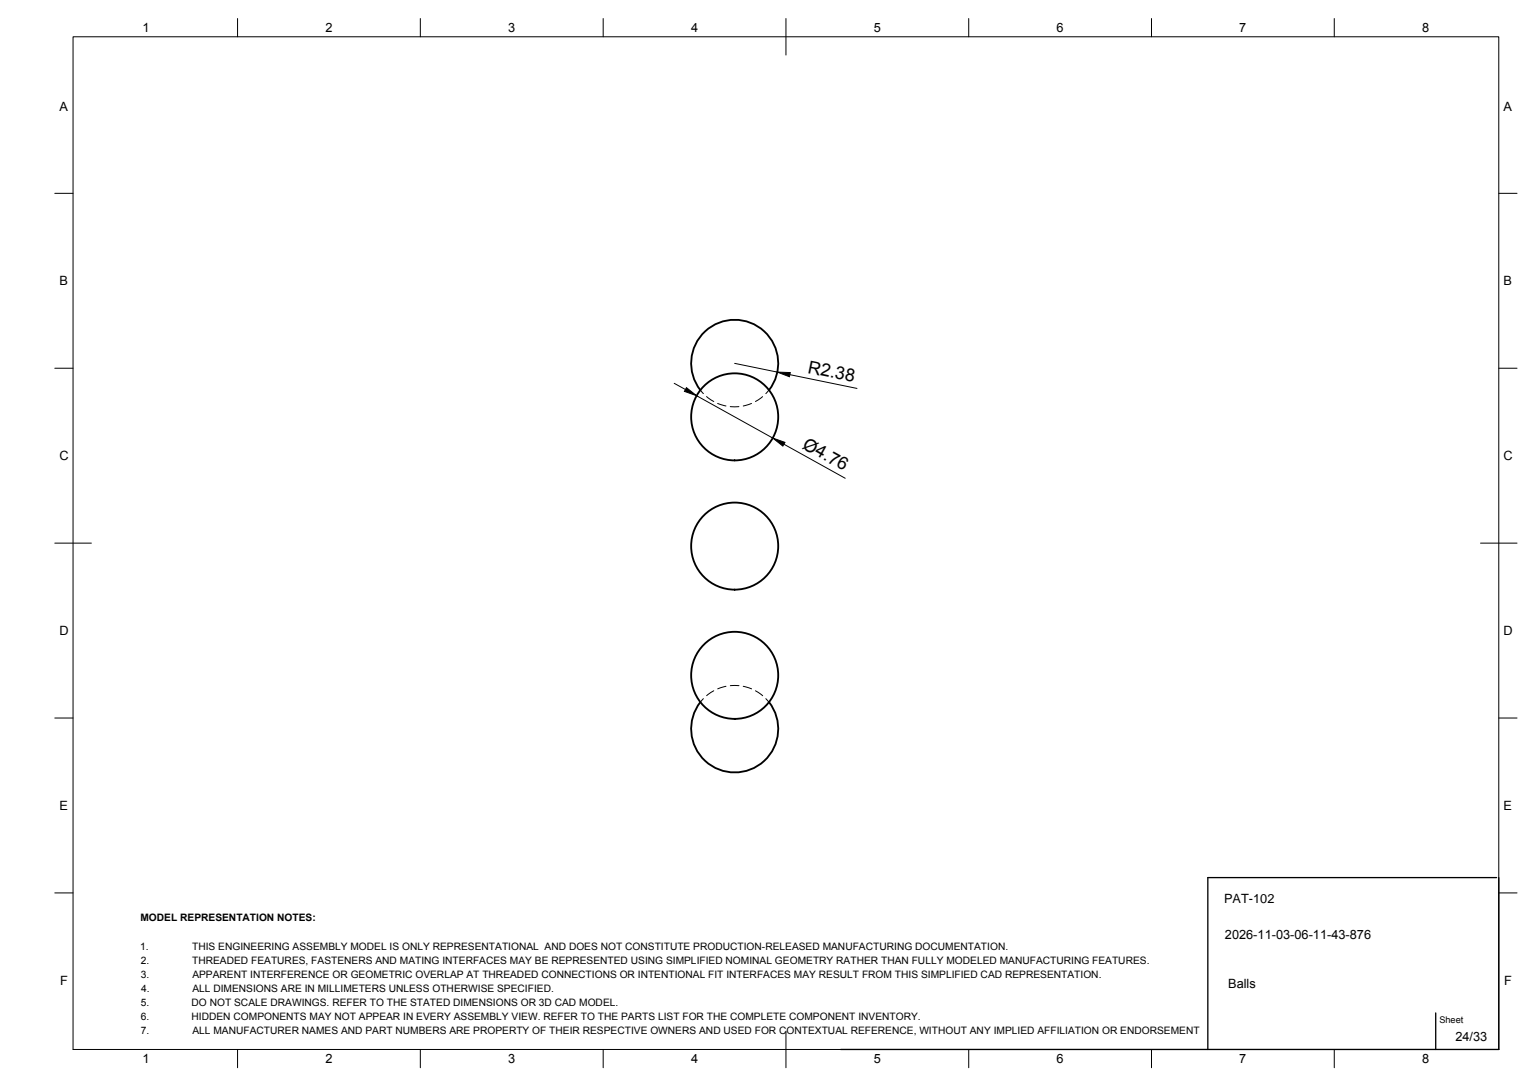
ISO-10303-21;
HEADER;
/* Generated by software containing ST-Developer
 * from STEP Tools, Inc. (www.steptools.com) 
 */

FILE_DESCRIPTION(
/* description */ ('Swing-away clamp arm'),
/* implementation_level */ '2;1');

FILE_NAME(
/* name */ 'Balls.step',
/* time_stamp */ '2026-10-28T03:26:03-07:00',
/* author */ (''),
/* organization */ (''),
/* preprocessor_version */ 'ST-DEVELOPER v20.2',
/* originating_system */ 'Autodesk Translation Framework v15.17.0.0',
/* authorisation */ '');

FILE_SCHEMA (('AUTOMOTIVE_DESIGN { 1 0 10303 214 3 1 1 }'));
ENDSEC;

DATA;
#10=MECHANICAL_DESIGN_GEOMETRIC_PRESENTATION_REPRESENTATION('',(#309,#310,#311,#312,#313,#314,#315,#316),#10627);
#11=SPHERICAL_SURFACE('',#5621,0.23815);
#12=SPHERICAL_SURFACE('',#5623,0.23815);
#13=SPHERICAL_SURFACE('',#5625,0.23815);
#14=SPHERICAL_SURFACE('',#5627,0.23815);
#15=SPHERICAL_SURFACE('',#5629,0.23815);
#16=SPHERICAL_SURFACE('',#5631,0.23815);
#17=SPHERICAL_SURFACE('',#5633,0.23815);
#18=SPHERICAL_SURFACE('',#5635,0.23815);
#257=SHAPE_REPRESENTATION_RELATIONSHIP('SRR','None',#10757,#283);
#283=ADVANCED_BREP_SHAPE_REPRESENTATION('',(#342,#343,#344,#345,#346,#347,
#348,#349),#10616);
#309=STYLED_ITEM('',(#10965),#342);
#310=STYLED_ITEM('',(#10965),#343);
#311=STYLED_ITEM('',(#10965),#344);
#312=STYLED_ITEM('',(#10965),#345);
#313=STYLED_ITEM('',(#10965),#346);
#314=STYLED_ITEM('',(#10965),#347);
#315=STYLED_ITEM('',(#10965),#348);
#316=STYLED_ITEM('',(#10965),#349);
#342=MANIFOLD_SOLID_BREP('Body1',#4916);
#343=MANIFOLD_SOLID_BREP('Body2',#4917);
#344=MANIFOLD_SOLID_BREP('Body3',#4918);
#345=MANIFOLD_SOLID_BREP('Body4',#4919);
#346=MANIFOLD_SOLID_BREP('Body5',#4920);
#347=MANIFOLD_SOLID_BREP('Body6',#4921);
#348=MANIFOLD_SOLID_BREP('Body7',#4922);
#349=MANIFOLD_SOLID_BREP('Body8',#4923);
#839=FACE_OUTER_BOUND('',#1224,.T.);
#840=FACE_OUTER_BOUND('',#1225,.T.);
#841=FACE_OUTER_BOUND('',#1226,.T.);
#842=FACE_OUTER_BOUND('',#1227,.T.);
#843=FACE_OUTER_BOUND('',#1228,.T.);
#844=FACE_OUTER_BOUND('',#1229,.T.);
#845=FACE_OUTER_BOUND('',#1230,.T.);
#846=FACE_OUTER_BOUND('',#1231,.T.);
#1224=EDGE_LOOP('',(#4105,#4106));
#1225=EDGE_LOOP('',(#4107,#4108));
#1226=EDGE_LOOP('',(#4109,#4110));
#1227=EDGE_LOOP('',(#4111,#4112));
#1228=EDGE_LOOP('',(#4113,#4114));
#1229=EDGE_LOOP('',(#4115,#4116));
#1230=EDGE_LOOP('',(#4117,#4118));
#1231=EDGE_LOOP('',(#4119,#4120));
#2161=CIRCLE('',#5622,0.23815);
#2162=CIRCLE('',#5624,0.23815);
#2163=CIRCLE('',#5626,0.23815);
#2164=CIRCLE('',#5628,0.23815);
#2165=CIRCLE('',#5630,0.23815);
#2166=CIRCLE('',#5632,0.23815);
#2167=CIRCLE('',#5634,0.23815);
#2168=CIRCLE('',#5636,0.23815);
#2534=VERTEX_POINT('',#9744);
#2535=VERTEX_POINT('',#9745);
#2536=VERTEX_POINT('',#9748);
#2537=VERTEX_POINT('',#9749);
#2538=VERTEX_POINT('',#9752);
#2539=VERTEX_POINT('',#9753);
#2540=VERTEX_POINT('',#9756);
#2541=VERTEX_POINT('',#9757);
#2542=VERTEX_POINT('',#9760);
#2543=VERTEX_POINT('',#9761);
#2544=VERTEX_POINT('',#9764);
#2545=VERTEX_POINT('',#9765);
#2546=VERTEX_POINT('',#9768);
#2547=VERTEX_POINT('',#9769);
#2548=VERTEX_POINT('',#9772);
#2549=VERTEX_POINT('',#9773);
#3085=EDGE_CURVE('',#2534,#2535,#2161,.T.);
#3086=EDGE_CURVE('',#2536,#2537,#2162,.T.);
#3087=EDGE_CURVE('',#2538,#2539,#2163,.T.);
#3088=EDGE_CURVE('',#2540,#2541,#2164,.T.);
#3089=EDGE_CURVE('',#2542,#2543,#2165,.T.);
#3090=EDGE_CURVE('',#2544,#2545,#2166,.T.);
#3091=EDGE_CURVE('',#2546,#2547,#2167,.T.);
#3092=EDGE_CURVE('',#2548,#2549,#2168,.T.);
#4105=ORIENTED_EDGE('',*,*,#3085,.T.);
#4106=ORIENTED_EDGE('',*,*,#3085,.F.);
#4107=ORIENTED_EDGE('',*,*,#3086,.T.);
#4108=ORIENTED_EDGE('',*,*,#3086,.F.);
#4109=ORIENTED_EDGE('',*,*,#3087,.T.);
#4110=ORIENTED_EDGE('',*,*,#3087,.F.);
#4111=ORIENTED_EDGE('',*,*,#3088,.T.);
#4112=ORIENTED_EDGE('',*,*,#3088,.F.);
#4113=ORIENTED_EDGE('',*,*,#3089,.T.);
#4114=ORIENTED_EDGE('',*,*,#3089,.F.);
#4115=ORIENTED_EDGE('',*,*,#3090,.T.);
#4116=ORIENTED_EDGE('',*,*,#3090,.F.);
#4117=ORIENTED_EDGE('',*,*,#3091,.T.);
#4118=ORIENTED_EDGE('',*,*,#3091,.F.);
#4119=ORIENTED_EDGE('',*,*,#3092,.T.);
#4120=ORIENTED_EDGE('',*,*,#3092,.F.);
#4794=ADVANCED_FACE('',(#839),#11,.T.);
#4795=ADVANCED_FACE('',(#840),#12,.T.);
#4796=ADVANCED_FACE('',(#841),#13,.T.);
#4797=ADVANCED_FACE('',(#842),#14,.T.);
#4798=ADVANCED_FACE('',(#843),#15,.T.);
#4799=ADVANCED_FACE('',(#844),#16,.T.);
#4800=ADVANCED_FACE('',(#845),#17,.T.);
#4801=ADVANCED_FACE('',(#846),#18,.T.);
#4916=CLOSED_SHELL('',(#4794));
#4917=CLOSED_SHELL('',(#4795));
#4918=CLOSED_SHELL('',(#4796));
#4919=CLOSED_SHELL('',(#4797));
#4920=CLOSED_SHELL('',(#4798));
#4921=CLOSED_SHELL('',(#4799));
#4922=CLOSED_SHELL('',(#4800));
#4923=CLOSED_SHELL('',(#4801));
#5620=AXIS2_PLACEMENT_3D('',#9742,#6909,#6910);
#5621=AXIS2_PLACEMENT_3D('',#9743,#6911,#6912);
#5622=AXIS2_PLACEMENT_3D('',#9746,#6913,#6914);
#5623=AXIS2_PLACEMENT_3D('',#9747,#6915,#6916);
#5624=AXIS2_PLACEMENT_3D('',#9750,#6917,#6918);
#5625=AXIS2_PLACEMENT_3D('',#9751,#6919,#6920);
#5626=AXIS2_PLACEMENT_3D('',#9754,#6921,#6922);
#5627=AXIS2_PLACEMENT_3D('',#9755,#6923,#6924);
#5628=AXIS2_PLACEMENT_3D('',#9758,#6925,#6926);
#5629=AXIS2_PLACEMENT_3D('',#9759,#6927,#6928);
#5630=AXIS2_PLACEMENT_3D('',#9762,#6929,#6930);
#5631=AXIS2_PLACEMENT_3D('',#9763,#6931,#6932);
#5632=AXIS2_PLACEMENT_3D('',#9766,#6933,#6934);
#5633=AXIS2_PLACEMENT_3D('',#9767,#6935,#6936);
#5634=AXIS2_PLACEMENT_3D('',#9770,#6937,#6938);
#5635=AXIS2_PLACEMENT_3D('',#9771,#6939,#6940);
#5636=AXIS2_PLACEMENT_3D('',#9774,#6941,#6942);
#6909=DIRECTION('axis',(0.,0.,1.));
#6910=DIRECTION('refdir',(1.,0.,0.));
#6911=DIRECTION('center_axis',(0.,0.,1.));
#6912=DIRECTION('ref_axis',(1.,0.,0.));
#6913=DIRECTION('center_axis',(1.22464679914735E-16,-1.,0.));
#6914=DIRECTION('ref_axis',(-1.,-1.22464679914735E-16,0.));
#6915=DIRECTION('center_axis',(0.707106781186548,0.,0.707106781186548));
#6916=DIRECTION('ref_axis',(0.707106781186548,0.,-0.707106781186548));
#6917=DIRECTION('center_axis',(8.65956056235494E-17,-1.,-8.65956056235493E-17));
#6918=DIRECTION('ref_axis',(-0.707106781186547,-1.22464679914735E-16,0.707106781186547));
#6919=DIRECTION('center_axis',(1.,0.,0.));
#6920=DIRECTION('ref_axis',(6.12323399573676E-17,0.,-1.));
#6921=DIRECTION('center_axis',(7.49879891330929E-33,-1.,-1.22464679914735E-16));
#6922=DIRECTION('ref_axis',(-6.12323399573676E-17,-1.22464679914735E-16,
1.));
#6923=DIRECTION('center_axis',(0.707106781186548,0.,-0.707106781186548));
#6924=DIRECTION('ref_axis',(-0.707106781186548,0.,-0.707106781186548));
#6925=DIRECTION('center_axis',(-8.65956056235493E-17,-1.,-8.65956056235494E-17));
#6926=DIRECTION('ref_axis',(0.707106781186547,-1.22464679914735E-16,0.707106781186547));
#6927=DIRECTION('center_axis',(0.,0.,-1.));
#6928=DIRECTION('ref_axis',(-1.,0.,-1.22464679914735E-16));
#6929=DIRECTION('center_axis',(-1.22464679914735E-16,-1.,-1.49975978266186E-32));
#6930=DIRECTION('ref_axis',(1.,-1.22464679914735E-16,1.22464679914735E-16));
#6931=DIRECTION('center_axis',(-0.707106781186547,0.,-0.707106781186548));
#6932=DIRECTION('ref_axis',(-0.707106781186548,0.,0.707106781186547));
#6933=DIRECTION('center_axis',(-8.65956056235493E-17,-1.,8.65956056235493E-17));
#6934=DIRECTION('ref_axis',(0.707106781186548,-1.22464679914735E-16,-0.707106781186547));
#6935=DIRECTION('center_axis',(-1.,0.,0.));
#6936=DIRECTION('ref_axis',(-1.83697019872103E-16,0.,1.));
#6937=DIRECTION('center_axis',(-2.24963967399279E-32,-1.,1.22464679914735E-16));
#6938=DIRECTION('ref_axis',(1.83697019872103E-16,-1.22464679914735E-16,
-1.));
#6939=DIRECTION('center_axis',(-0.707106781186548,0.,0.707106781186548));
#6940=DIRECTION('ref_axis',(0.707106781186547,0.,0.707106781186548));
#6941=DIRECTION('center_axis',(8.65956056235493E-17,-1.,8.65956056235493E-17));
#6942=DIRECTION('ref_axis',(-0.707106781186547,-1.22464679914735E-16,-0.707106781186548));
#9742=CARTESIAN_POINT('',(0.,0.,0.));
#9743=CARTESIAN_POINT('Origin',(1.,0.,0.));
#9744=CARTESIAN_POINT('',(1.,-1.78583896120461E-33,0.23815));
#9745=CARTESIAN_POINT('',(1.,-1.78583896120461E-33,-0.23815));
#9746=CARTESIAN_POINT('Origin',(1.,0.,0.));
#9747=CARTESIAN_POINT('Origin',(0.707106781186548,0.,-0.707106781186547));
#9748=CARTESIAN_POINT('',(0.875504261126124,-1.78583896120461E-33,-0.538709301246971));
#9749=CARTESIAN_POINT('',(0.538709301246971,-1.78583896120461E-33,-0.875504261126124));
#9750=CARTESIAN_POINT('Origin',(0.707106781186548,0.,-0.707106781186547));
#9751=CARTESIAN_POINT('Origin',(6.12323399573677E-17,0.,-1.));
#9752=CARTESIAN_POINT('',(0.23815,-1.78583896120461E-33,-1.));
#9753=CARTESIAN_POINT('',(-0.23815,-1.78583896120461E-33,-1.));
#9754=CARTESIAN_POINT('Origin',(6.12323399573677E-17,0.,-1.));
#9755=CARTESIAN_POINT('Origin',(-0.707106781186547,0.,-0.707106781186548));
#9756=CARTESIAN_POINT('',(-0.538709301246971,-1.78583896120461E-33,-0.875504261126124));
#9757=CARTESIAN_POINT('',(-0.875504261126124,-1.78583896120461E-33,-0.538709301246971));
#9758=CARTESIAN_POINT('Origin',(-0.707106781186547,0.,-0.707106781186548));
#9759=CARTESIAN_POINT('Origin',(-1.,0.,-1.22464679914735E-16));
#9760=CARTESIAN_POINT('',(-1.,-1.78583896120461E-33,-0.23815));
#9761=CARTESIAN_POINT('',(-1.,-1.78583896120461E-33,0.23815));
#9762=CARTESIAN_POINT('Origin',(-1.,0.,-1.22464679914735E-16));
#9763=CARTESIAN_POINT('Origin',(-0.707106781186548,0.,0.707106781186547));
#9764=CARTESIAN_POINT('',(-0.875504261126124,-7.94881478324376E-33,0.538709301246971));
#9765=CARTESIAN_POINT('',(-0.538709301246971,4.37713686083455E-33,0.875504261126124));
#9766=CARTESIAN_POINT('Origin',(-0.707106781186548,0.,0.707106781186547));
#9767=CARTESIAN_POINT('Origin',(-1.83697019872103E-16,0.,1.));
#9768=CARTESIAN_POINT('',(-0.23815,-1.78583896120461E-33,1.));
#9769=CARTESIAN_POINT('',(0.23815,-1.78583896120461E-33,1.));
#9770=CARTESIAN_POINT('Origin',(-1.83697019872103E-16,0.,1.));
#9771=CARTESIAN_POINT('Origin',(0.707106781186547,0.,0.707106781186548));
#9772=CARTESIAN_POINT('',(0.538709301246971,-4.86732687222419E-33,0.875504261126124));
#9773=CARTESIAN_POINT('',(0.875504261126124,1.29564894981497E-33,0.538709301246971));
#9774=CARTESIAN_POINT('Origin',(0.707106781186547,0.,0.707106781186548));
#10584=UNCERTAINTY_MEASURE_WITH_UNIT(LENGTH_MEASURE(0.001),#10628,
'DISTANCE_ACCURACY_VALUE',
'Maximum model space distance between geometric entities at asserted c
onnectivities');
#10595=UNCERTAINTY_MEASURE_WITH_UNIT(LENGTH_MEASURE(0.001),#10628,
'DISTANCE_ACCURACY_VALUE',
'Maximum model space distance between geometric entities at asserted c
onnectivities');
#10616=(
GEOMETRIC_REPRESENTATION_CONTEXT(3)
GLOBAL_UNCERTAINTY_ASSIGNED_CONTEXT((#10584))
GLOBAL_UNIT_ASSIGNED_CONTEXT((#10628,#10630,#10631))
REPRESENTATION_CONTEXT('','3D')
);
#10627=(
GEOMETRIC_REPRESENTATION_CONTEXT(3)
GLOBAL_UNCERTAINTY_ASSIGNED_CONTEXT((#10595))
GLOBAL_UNIT_ASSIGNED_CONTEXT((#10628,#10630,#10631))
REPRESENTATION_CONTEXT('','3D')
);
#10628=(
LENGTH_UNIT()
NAMED_UNIT(*)
SI_UNIT(.CENTI.,.METRE.)
);
#10630=(
NAMED_UNIT(*)
PLANE_ANGLE_UNIT()
SI_UNIT($,.RADIAN.)
);
#10631=(
NAMED_UNIT(*)
SI_UNIT($,.STERADIAN.)
SOLID_ANGLE_UNIT()
);
#10652=SHAPE_DEFINITION_REPRESENTATION(#10693,#10757);
#10693=PRODUCT_DEFINITION_SHAPE('',$,#10789);
#10757=SHAPE_REPRESENTATION('',(#5620),#10616);
#10768=PRODUCT_DEFINITION_CONTEXT('part definition',#10863,'design');
#10789=PRODUCT_DEFINITION('Balls','Balls',#10820,#10768);
#10820=PRODUCT_DEFINITION_FORMATION('',$,#10885);
#10863=APPLICATION_CONTEXT(
'Core Data for Automotive Mechanical Design Process');
#10864=PRODUCT_CONTEXT('part definition',#10863,'mechanical');
#10885=PRODUCT('Balls','Balls','Balls',(#10864));
#10959=COLOUR_RGB('Grey',0.48,0.52,0.57);
#10960=FILL_AREA_STYLE_COLOUR('',#10959);
#10961=FILL_AREA_STYLE('',(#10960));
#10962=SURFACE_STYLE_FILL_AREA(#10961);
#10963=SURFACE_SIDE_STYLE('',(#10962));
#10964=SURFACE_STYLE_USAGE(.BOTH.,#10963);
#10965=PRESENTATION_STYLE_ASSIGNMENT((#10964));
ENDSEC;
END-ISO-10303-21;
